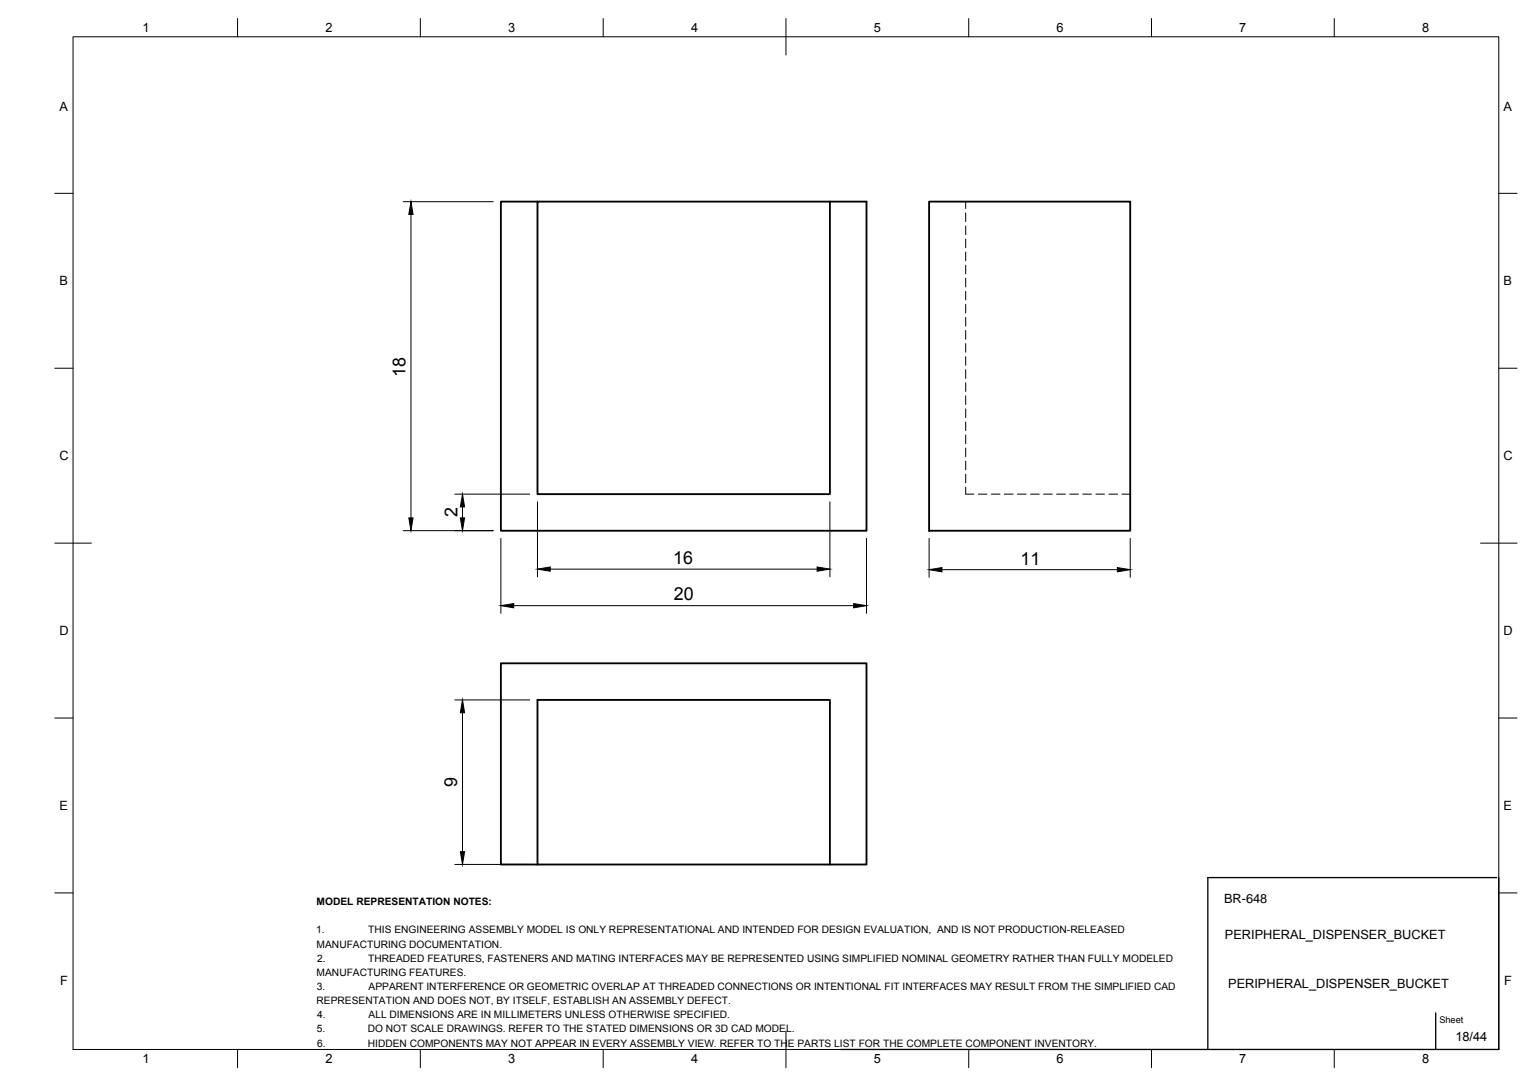
ISO-10303-21;
HEADER;
FILE_DESCRIPTION((''),'2;1');
FILE_NAME('PERIPHERAL_DISPENSER_BUCKET.step','2026-10-01T22:05:39-07:00',(''),(''),'','','');
FILE_SCHEMA (('AUTOMOTIVE_DESIGN { 1 0 10303 214 3 1 1 }'));
ENDSEC;
DATA;
#10=MECHANICAL_DESIGN_GEOMETRIC_PRESENTATION_REPRESENTATION('',(#618),#24628);
#534=SHAPE_REPRESENTATION_RELATIONSHIP('SRR','None',#24806,#576) ;
#576=ADVANCED_BREP_SHAPE_REPRESENTATION('',(#658),#24596) ;
#618=STYLED_ITEM('',(#25036),#658) ;
#658=MANIFOLD_SOLID_BREP('PERIPHERAL_DISPENSER_BUCKET',#13129) ;
#1305=LINE('',#21077,#2141) ;
#1306=LINE('',#21079,#2142) ;
#1307=LINE('',#21081,#2143) ;
#1308=LINE('',#21082,#2144) ;
#1309=LINE('',#21085,#2145) ;
#1310=LINE('',#21087,#2146) ;
#1311=LINE('',#21088,#2147) ;
#1312=LINE('',#21091,#2148) ;
#1313=LINE('',#21092,#2149) ;
#1314=LINE('',#21095,#2150) ;
#1315=LINE('',#21096,#2151) ;
#1316=LINE('',#21099,#2152) ;
#1317=LINE('',#21101,#2153) ;
#1318=LINE('',#21103,#2154) ;
#1319=LINE('',#21105,#2155) ;
#1320=LINE('',#21106,#2156) ;
#1321=LINE('',#21109,#2157) ;
#1322=LINE('',#21111,#2158) ;
#1323=LINE('',#21112,#2159) ;
#1324=LINE('',#21115,#2160) ;
#1325=LINE('',#21117,#2161) ;
#1326=LINE('',#21118,#2162) ;
#1327=LINE('',#21120,#2163) ;
#1328=LINE('',#21121,#2164) ;
#2141=VECTOR('',#16826,1.) ;
#2142=VECTOR('',#16827,1.) ;
#2143=VECTOR('',#16828,1.) ;
#2144=VECTOR('',#16829,1.) ;
#2145=VECTOR('',#16832,1.) ;
#2146=VECTOR('',#16833,1.) ;
#2147=VECTOR('',#16834,1.) ;
#2148=VECTOR('',#16837,1.) ;
#2149=VECTOR('',#16838,1.) ;
#2150=VECTOR('',#16841,1.) ;
#2151=VECTOR('',#16842,1.) ;
#2152=VECTOR('',#16845,1.) ;
#2153=VECTOR('',#16846,1.) ;
#2154=VECTOR('',#16847,1.) ;
#2155=VECTOR('',#16848,1.) ;
#2156=VECTOR('',#16849,1.) ;
#2157=VECTOR('',#16852,1.) ;
#2158=VECTOR('',#16853,1.) ;
#2159=VECTOR('',#16854,1.) ;
#2160=VECTOR('',#16857,1.) ;
#2161=VECTOR('',#16858,1.) ;
#2162=VECTOR('',#16859,1.) ;
#2163=VECTOR('',#16862,1.) ;
#2164=VECTOR('',#16863,1.) ;
#3216=FACE_OUTER_BOUND('',#4151,.T.) ;
#3217=FACE_OUTER_BOUND('',#4152,.T.) ;
#3218=FACE_OUTER_BOUND('',#4153,.T.) ;
#3219=FACE_OUTER_BOUND('',#4154,.T.) ;
#3220=FACE_OUTER_BOUND('',#4155,.T.) ;
#3221=FACE_OUTER_BOUND('',#4156,.T.) ;
#3222=FACE_OUTER_BOUND('',#4157,.T.) ;
#3223=FACE_OUTER_BOUND('',#4158,.T.) ;
#3224=FACE_OUTER_BOUND('',#4159,.T.) ;
#3225=FACE_OUTER_BOUND('',#4160,.T.) ;
#4151=EDGE_LOOP('',(#9675,#9676,#9677,#9678)) ;
#4152=EDGE_LOOP('',(#9679,#9680,#9681,#9682)) ;
#4153=EDGE_LOOP('',(#9683,#9684,#9685,#9686)) ;
#4154=EDGE_LOOP('',(#9687,#9688,#9689,#9690)) ;
#4155=EDGE_LOOP('',(#9691,#9692,#9693,#9694,#9695,#9696,#9697,#9698)) ;
#4156=EDGE_LOOP('',(#9699,#9700,#9701,#9702,#9703,#9704,#9705,#9706)) ;
#4157=EDGE_LOOP('',(#9707,#9708,#9709,#9710)) ;
#4158=EDGE_LOOP('',(#9711,#9712,#9713,#9714)) ;
#4159=EDGE_LOOP('',(#9715,#9716,#9717,#9718)) ;
#4160=EDGE_LOOP('',(#9719,#9720,#9721,#9722)) ;
#5933=VERTEX_POINT('',#21075) ;
#5934=VERTEX_POINT('',#21076) ;
#5935=VERTEX_POINT('',#21078) ;
#5936=VERTEX_POINT('',#21080) ;
#5937=VERTEX_POINT('',#21084) ;
#5938=VERTEX_POINT('',#21086) ;
#5939=VERTEX_POINT('',#21090) ;
#5940=VERTEX_POINT('',#21094) ;
#5941=VERTEX_POINT('',#21098) ;
#5942=VERTEX_POINT('',#21100) ;
#5943=VERTEX_POINT('',#21102) ;
#5944=VERTEX_POINT('',#21104) ;
#5945=VERTEX_POINT('',#21108) ;
#5946=VERTEX_POINT('',#21110) ;
#5947=VERTEX_POINT('',#21114) ;
#5948=VERTEX_POINT('',#21116) ;
#7327=EDGE_CURVE('',#5933,#5934,#1305,.T.) ;
#7328=EDGE_CURVE('',#5935,#5933,#1306,.T.) ;
#7329=EDGE_CURVE('',#5936,#5935,#1307,.T.) ;
#7330=EDGE_CURVE('',#5934,#5936,#1308,.T.) ;
#7331=EDGE_CURVE('',#5934,#5937,#1309,.T.) ;
#7332=EDGE_CURVE('',#5938,#5936,#1310,.T.) ;
#7333=EDGE_CURVE('',#5937,#5938,#1311,.T.) ;
#7334=EDGE_CURVE('',#5938,#5939,#1312,.T.) ;
#7335=EDGE_CURVE('',#5939,#5935,#1313,.T.) ;
#7336=EDGE_CURVE('',#5940,#5933,#1314,.T.) ;
#7337=EDGE_CURVE('',#5939,#5940,#1315,.T.) ;
#7338=EDGE_CURVE('',#5941,#5937,#1316,.T.) ;
#7339=EDGE_CURVE('',#5941,#5942,#1317,.T.) ;
#7340=EDGE_CURVE('',#5943,#5942,#1318,.T.) ;
#7341=EDGE_CURVE('',#5944,#5943,#1319,.T.) ;
#7342=EDGE_CURVE('',#5940,#5944,#1320,.T.) ;
#7343=EDGE_CURVE('',#5944,#5945,#1321,.T.) ;
#7344=EDGE_CURVE('',#5945,#5946,#1322,.T.) ;
#7345=EDGE_CURVE('',#5946,#5941,#1323,.T.) ;
#7346=EDGE_CURVE('',#5942,#5947,#1324,.T.) ;
#7347=EDGE_CURVE('',#5947,#5948,#1325,.T.) ;
#7348=EDGE_CURVE('',#5948,#5943,#1326,.T.) ;
#7349=EDGE_CURVE('',#5945,#5948,#1327,.T.) ;
#7350=EDGE_CURVE('',#5946,#5947,#1328,.T.) ;
#9675=ORIENTED_EDGE('',*,*,#7327,.F.) ;
#9676=ORIENTED_EDGE('',*,*,#7328,.F.) ;
#9677=ORIENTED_EDGE('',*,*,#7329,.F.) ;
#9678=ORIENTED_EDGE('',*,*,#7330,.F.) ;
#9679=ORIENTED_EDGE('',*,*,#7331,.F.) ;
#9680=ORIENTED_EDGE('',*,*,#7330,.T.) ;
#9681=ORIENTED_EDGE('',*,*,#7332,.F.) ;
#9682=ORIENTED_EDGE('',*,*,#7333,.F.) ;
#9683=ORIENTED_EDGE('',*,*,#7334,.F.) ;
#9684=ORIENTED_EDGE('',*,*,#7332,.T.) ;
#9685=ORIENTED_EDGE('',*,*,#7329,.T.) ;
#9686=ORIENTED_EDGE('',*,*,#7335,.F.) ;
#9687=ORIENTED_EDGE('',*,*,#7336,.F.) ;
#9688=ORIENTED_EDGE('',*,*,#7337,.F.) ;
#9689=ORIENTED_EDGE('',*,*,#7335,.T.) ;
#9690=ORIENTED_EDGE('',*,*,#7328,.T.) ;
#9691=ORIENTED_EDGE('',*,*,#7336,.T.) ;
#9692=ORIENTED_EDGE('',*,*,#7327,.T.) ;
#9693=ORIENTED_EDGE('',*,*,#7331,.T.) ;
#9694=ORIENTED_EDGE('',*,*,#7338,.F.) ;
#9695=ORIENTED_EDGE('',*,*,#7339,.T.) ;
#9696=ORIENTED_EDGE('',*,*,#7340,.F.) ;
#9697=ORIENTED_EDGE('',*,*,#7341,.F.) ;
#9698=ORIENTED_EDGE('',*,*,#7342,.F.) ;
#9699=ORIENTED_EDGE('',*,*,#7337,.T.) ;
#9700=ORIENTED_EDGE('',*,*,#7342,.T.) ;
#9701=ORIENTED_EDGE('',*,*,#7343,.T.) ;
#9702=ORIENTED_EDGE('',*,*,#7344,.T.) ;
#9703=ORIENTED_EDGE('',*,*,#7345,.T.) ;
#9704=ORIENTED_EDGE('',*,*,#7338,.T.) ;
#9705=ORIENTED_EDGE('',*,*,#7333,.T.) ;
#9706=ORIENTED_EDGE('',*,*,#7334,.T.) ;
#9707=ORIENTED_EDGE('',*,*,#7346,.T.) ;
#9708=ORIENTED_EDGE('',*,*,#7347,.T.) ;
#9709=ORIENTED_EDGE('',*,*,#7348,.T.) ;
#9710=ORIENTED_EDGE('',*,*,#7340,.T.) ;
#9711=ORIENTED_EDGE('',*,*,#7349,.T.) ;
#9712=ORIENTED_EDGE('',*,*,#7347,.F.) ;
#9713=ORIENTED_EDGE('',*,*,#7350,.F.) ;
#9714=ORIENTED_EDGE('',*,*,#7344,.F.) ;
#9715=ORIENTED_EDGE('',*,*,#7341,.T.) ;
#9716=ORIENTED_EDGE('',*,*,#7348,.F.) ;
#9717=ORIENTED_EDGE('',*,*,#7349,.F.) ;
#9718=ORIENTED_EDGE('',*,*,#7343,.F.) ;
#9719=ORIENTED_EDGE('',*,*,#7350,.T.) ;
#9720=ORIENTED_EDGE('',*,*,#7346,.F.) ;
#9721=ORIENTED_EDGE('',*,*,#7339,.F.) ;
#9722=ORIENTED_EDGE('',*,*,#7345,.F.) ;
#12126=PLANE('',#14217) ;
#12127=PLANE('',#14218) ;
#12128=PLANE('',#14219) ;
#12129=PLANE('',#14220) ;
#12130=PLANE('',#14221) ;
#12131=PLANE('',#14222) ;
#12132=PLANE('',#14223) ;
#12133=PLANE('',#14224) ;
#12134=PLANE('',#14225) ;
#12135=PLANE('',#14226) ;
#12611=ADVANCED_FACE('',(#3216),#12126,.T.) ;
#12612=ADVANCED_FACE('',(#3217),#12127,.T.) ;
#12613=ADVANCED_FACE('',(#3218),#12128,.T.) ;
#12614=ADVANCED_FACE('',(#3219),#12129,.T.) ;
#12615=ADVANCED_FACE('',(#3220),#12130,.F.) ;
#12616=ADVANCED_FACE('',(#3221),#12131,.T.) ;
#12617=ADVANCED_FACE('',(#3222),#12132,.F.) ;
#12618=ADVANCED_FACE('',(#3223),#12133,.F.) ;
#12619=ADVANCED_FACE('',(#3224),#12134,.F.) ;
#12620=ADVANCED_FACE('',(#3225),#12135,.F.) ;
#13129=CLOSED_SHELL('',(#12611,#12612,#12613,#12614,#12615,#12616,#12617,
#12618,#12619,#12620)) ;
#14216=AXIS2_PLACEMENT_3D('',#21073,#16822,#16823) ;
#14217=AXIS2_PLACEMENT_3D('',#21074,#16824,#16825) ;
#14218=AXIS2_PLACEMENT_3D('',#21083,#16830,#16831) ;
#14219=AXIS2_PLACEMENT_3D('',#21089,#16835,#16836) ;
#14220=AXIS2_PLACEMENT_3D('',#21093,#16839,#16840) ;
#14221=AXIS2_PLACEMENT_3D('',#21097,#16843,#16844) ;
#14222=AXIS2_PLACEMENT_3D('',#21107,#16850,#16851) ;
#14223=AXIS2_PLACEMENT_3D('',#21113,#16855,#16856) ;
#14224=AXIS2_PLACEMENT_3D('',#21119,#16860,#16861) ;
#14225=AXIS2_PLACEMENT_3D('',#21122,#16864,#16865) ;
#14226=AXIS2_PLACEMENT_3D('',#21123,#16866,#16867) ;
#16822=DIRECTION('axis',(0.,0.,1.)) ;
#16823=DIRECTION('refdir',(1.,0.,0.)) ;
#16824=DIRECTION('center_axis',(0.,0.,1.)) ;
#16825=DIRECTION('ref_axis',(1.,0.,0.)) ;
#16826=DIRECTION('',(1.,0.,0.)) ;
#16827=DIRECTION('',(0.,1.,0.)) ;
#16828=DIRECTION('',(-1.,0.,0.)) ;
#16829=DIRECTION('',(0.,-1.,0.)) ;
#16830=DIRECTION('center_axis',(-1.,0.,0.)) ;
#16831=DIRECTION('ref_axis',(0.,0.,1.)) ;
#16832=DIRECTION('',(0.,0.,1.)) ;
#16833=DIRECTION('',(0.,0.,-1.)) ;
#16834=DIRECTION('',(0.,-1.,0.)) ;
#16835=DIRECTION('center_axis',(0.,1.,0.)) ;
#16836=DIRECTION('ref_axis',(0.,0.,1.)) ;
#16837=DIRECTION('',(-1.,0.,0.)) ;
#16838=DIRECTION('',(0.,0.,-1.)) ;
#16839=DIRECTION('center_axis',(1.,0.,0.)) ;
#16840=DIRECTION('ref_axis',(0.,0.,-1.)) ;
#16841=DIRECTION('',(0.,0.,-1.)) ;
#16842=DIRECTION('',(0.,1.,0.)) ;
#16843=DIRECTION('center_axis',(0.,-1.,0.)) ;
#16844=DIRECTION('ref_axis',(0.,0.,-1.)) ;
#16845=DIRECTION('',(-1.,0.,0.)) ;
#16846=DIRECTION('',(0.,0.,-1.)) ;
#16847=DIRECTION('',(1.,0.,0.)) ;
#16848=DIRECTION('',(0.,0.,-1.)) ;
#16849=DIRECTION('',(-1.,0.,0.)) ;
#16850=DIRECTION('center_axis',(0.,0.,1.)) ;
#16851=DIRECTION('ref_axis',(1.,0.,0.)) ;
#16852=DIRECTION('',(0.,-1.,0.)) ;
#16853=DIRECTION('',(1.,0.,0.)) ;
#16854=DIRECTION('',(0.,1.,0.)) ;
#16855=DIRECTION('center_axis',(0.,0.,1.)) ;
#16856=DIRECTION('ref_axis',(1.,0.,0.)) ;
#16857=DIRECTION('',(0.,-1.,0.)) ;
#16858=DIRECTION('',(-1.,0.,0.)) ;
#16859=DIRECTION('',(0.,1.,0.)) ;
#16860=DIRECTION('center_axis',(0.,1.,0.)) ;
#16861=DIRECTION('ref_axis',(0.,0.,1.)) ;
#16862=DIRECTION('',(0.,0.,-1.)) ;
#16863=DIRECTION('',(0.,0.,-1.)) ;
#16864=DIRECTION('center_axis',(1.,0.,0.)) ;
#16865=DIRECTION('ref_axis',(0.,0.,-1.)) ;
#16866=DIRECTION('center_axis',(-1.,0.,0.)) ;
#16867=DIRECTION('ref_axis',(0.,0.,1.)) ;
#21073=CARTESIAN_POINT('',(0.,0.,0.)) ;
#21074=CARTESIAN_POINT('Origin',(0.,1.05,0.2)) ;
#21075=CARTESIAN_POINT('',(-0.8,1.8,0.2)) ;
#21076=CARTESIAN_POINT('',(0.8,1.8,0.2)) ;
#21077=CARTESIAN_POINT('',(0.,1.8,0.2)) ;
#21078=CARTESIAN_POINT('',(-0.8,0.2,0.2)) ;
#21079=CARTESIAN_POINT('',(-0.8,1.05,0.2)) ;
#21080=CARTESIAN_POINT('',(0.8,0.2,0.2)) ;
#21081=CARTESIAN_POINT('',(0.,0.2,0.2)) ;
#21082=CARTESIAN_POINT('',(0.8,1.05,0.2)) ;
#21083=CARTESIAN_POINT('Origin',(0.8,1.05,0.7)) ;
#21084=CARTESIAN_POINT('',(0.8,1.8,1.1)) ;
#21085=CARTESIAN_POINT('',(0.8,1.8,0.625)) ;
#21086=CARTESIAN_POINT('',(0.8,0.2,1.1)) ;
#21087=CARTESIAN_POINT('',(0.8,0.2,0.7)) ;
#21088=CARTESIAN_POINT('',(0.8,0.975,1.1)) ;
#21089=CARTESIAN_POINT('Origin',(0.,0.2,0.7)) ;
#21090=CARTESIAN_POINT('',(-0.8,0.2,1.1)) ;
#21091=CARTESIAN_POINT('',(0.,0.2,1.1)) ;
#21092=CARTESIAN_POINT('',(-0.8,0.2,0.7)) ;
#21093=CARTESIAN_POINT('Origin',(-0.8,1.05,0.7)) ;
#21094=CARTESIAN_POINT('',(-0.8,1.8,1.1)) ;
#21095=CARTESIAN_POINT('',(-0.8,1.8,0.625)) ;
#21096=CARTESIAN_POINT('',(-0.8,0.975,1.1)) ;
#21097=CARTESIAN_POINT('Origin',(0.,1.8,0.55)) ;
#21098=CARTESIAN_POINT('',(1.,1.8,1.1)) ;
#21099=CARTESIAN_POINT('',(0.,1.8,1.1)) ;
#21100=CARTESIAN_POINT('',(1.,1.8,0.)) ;
#21101=CARTESIAN_POINT('',(1.,1.8,0.55)) ;
#21102=CARTESIAN_POINT('',(-1.,1.8,0.)) ;
#21103=CARTESIAN_POINT('',(0.,1.8,0.)) ;
#21104=CARTESIAN_POINT('',(-1.,1.8,1.1)) ;
#21105=CARTESIAN_POINT('',(-1.,1.8,0.55)) ;
#21106=CARTESIAN_POINT('',(0.,1.8,1.1)) ;
#21107=CARTESIAN_POINT('Origin',(0.,0.9,1.1)) ;
#21108=CARTESIAN_POINT('',(-1.,0.,1.1)) ;
#21109=CARTESIAN_POINT('',(-1.,0.9,1.1)) ;
#21110=CARTESIAN_POINT('',(1.,0.,1.1)) ;
#21111=CARTESIAN_POINT('',(0.,0.,1.1)) ;
#21112=CARTESIAN_POINT('',(1.,0.9,1.1)) ;
#21113=CARTESIAN_POINT('Origin',(0.,0.9,0.)) ;
#21114=CARTESIAN_POINT('',(1.,0.,0.)) ;
#21115=CARTESIAN_POINT('',(1.,0.9,0.)) ;
#21116=CARTESIAN_POINT('',(-1.,0.,0.)) ;
#21117=CARTESIAN_POINT('',(0.,0.,0.)) ;
#21118=CARTESIAN_POINT('',(-1.,0.9,0.)) ;
#21119=CARTESIAN_POINT('Origin',(0.,0.,0.55)) ;
#21120=CARTESIAN_POINT('',(-1.,0.,0.55)) ;
#21121=CARTESIAN_POINT('',(1.,0.,0.55)) ;
#21122=CARTESIAN_POINT('Origin',(-1.,0.9,0.55)) ;
#21123=CARTESIAN_POINT('Origin',(1.,0.9,0.55)) ;
#24548=UNCERTAINTY_MEASURE_WITH_UNIT(LENGTH_MEASURE(0.001),#24629,
'DISTANCE_ACCURACY_VALUE',
'Maximum model space distance between geometric entities at asserted c
onnectivities') ;
#24580=UNCERTAINTY_MEASURE_WITH_UNIT(LENGTH_MEASURE(0.001),#24629,
'DISTANCE_ACCURACY_VALUE',
'Maximum model space distance between geometric entities at asserted c
onnectivities') ;
#24596=(
GEOMETRIC_REPRESENTATION_CONTEXT(3)
GLOBAL_UNCERTAINTY_ASSIGNED_CONTEXT((#24548))
GLOBAL_UNIT_ASSIGNED_CONTEXT((#24629,#24631,#24632))
REPRESENTATION_CONTEXT('','3D')
) ;
#24628=(
GEOMETRIC_REPRESENTATION_CONTEXT(3)
GLOBAL_UNCERTAINTY_ASSIGNED_CONTEXT((#24580))
GLOBAL_UNIT_ASSIGNED_CONTEXT((#24629,#24631,#24632))
REPRESENTATION_CONTEXT('','3D')
) ;
#24629=(
LENGTH_UNIT()
NAMED_UNIT(*)
SI_UNIT(.CENTI.,.METRE.)
) ;
#24631=(
NAMED_UNIT(*)
PLANE_ANGLE_UNIT()
SI_UNIT($,.RADIAN.)
) ;
#24632=(
NAMED_UNIT(*)
SI_UNIT($,.STERADIAN.)
SOLID_ANGLE_UNIT()
) ;
#24648=SHAPE_DEFINITION_REPRESENTATION(#24695,#24806) ;
#24695=PRODUCT_DEFINITION_SHAPE('',$,#24854) ;
#24806=SHAPE_REPRESENTATION('',(#14216),#24596) ;
#24838=PRODUCT_DEFINITION_CONTEXT('part definition',#24981,'design') ;
#24854=PRODUCT_DEFINITION('PERIPHERAL_DISPENSER_BUCKET',
'PERIPHERAL_DISPENSER_BUCKET',#24901,#24838) ;
#24901=PRODUCT_DEFINITION_FORMATION('',$,#24998) ;
#24981=APPLICATION_CONTEXT(
'Core Data for Automotive Mechanical Design Process') ;
#24982=PRODUCT_CONTEXT('part definition',#24981,'mechanical') ;
#24998=PRODUCT('PERIPHERAL_DISPENSER_BUCKET','PERIPHERAL_DISPENSER_BUCKET',
$,(#24982)) ;
#25036=PRESENTATION_STYLE_ASSIGNMENT((#25046)) ;
#25046=SURFACE_STYLE_USAGE(.BOTH.,#25056) ;
#25056=SURFACE_SIDE_STYLE('',(#25066)) ;
#25066=SURFACE_STYLE_FILL_AREA(#25076) ;
#25076=FILL_AREA_STYLE('Nylon 6-6 (White)',(#25086)) ;
#25086=FILL_AREA_STYLE_COLOUR('Nylon 6-6 (White)',#25096) ;
#25096=COLOUR_RGB('Nylon 6-6 (White)', 0.31764706, 0.68627451, 0.89019608) ;
ENDSEC;
END-ISO-10303-21;
